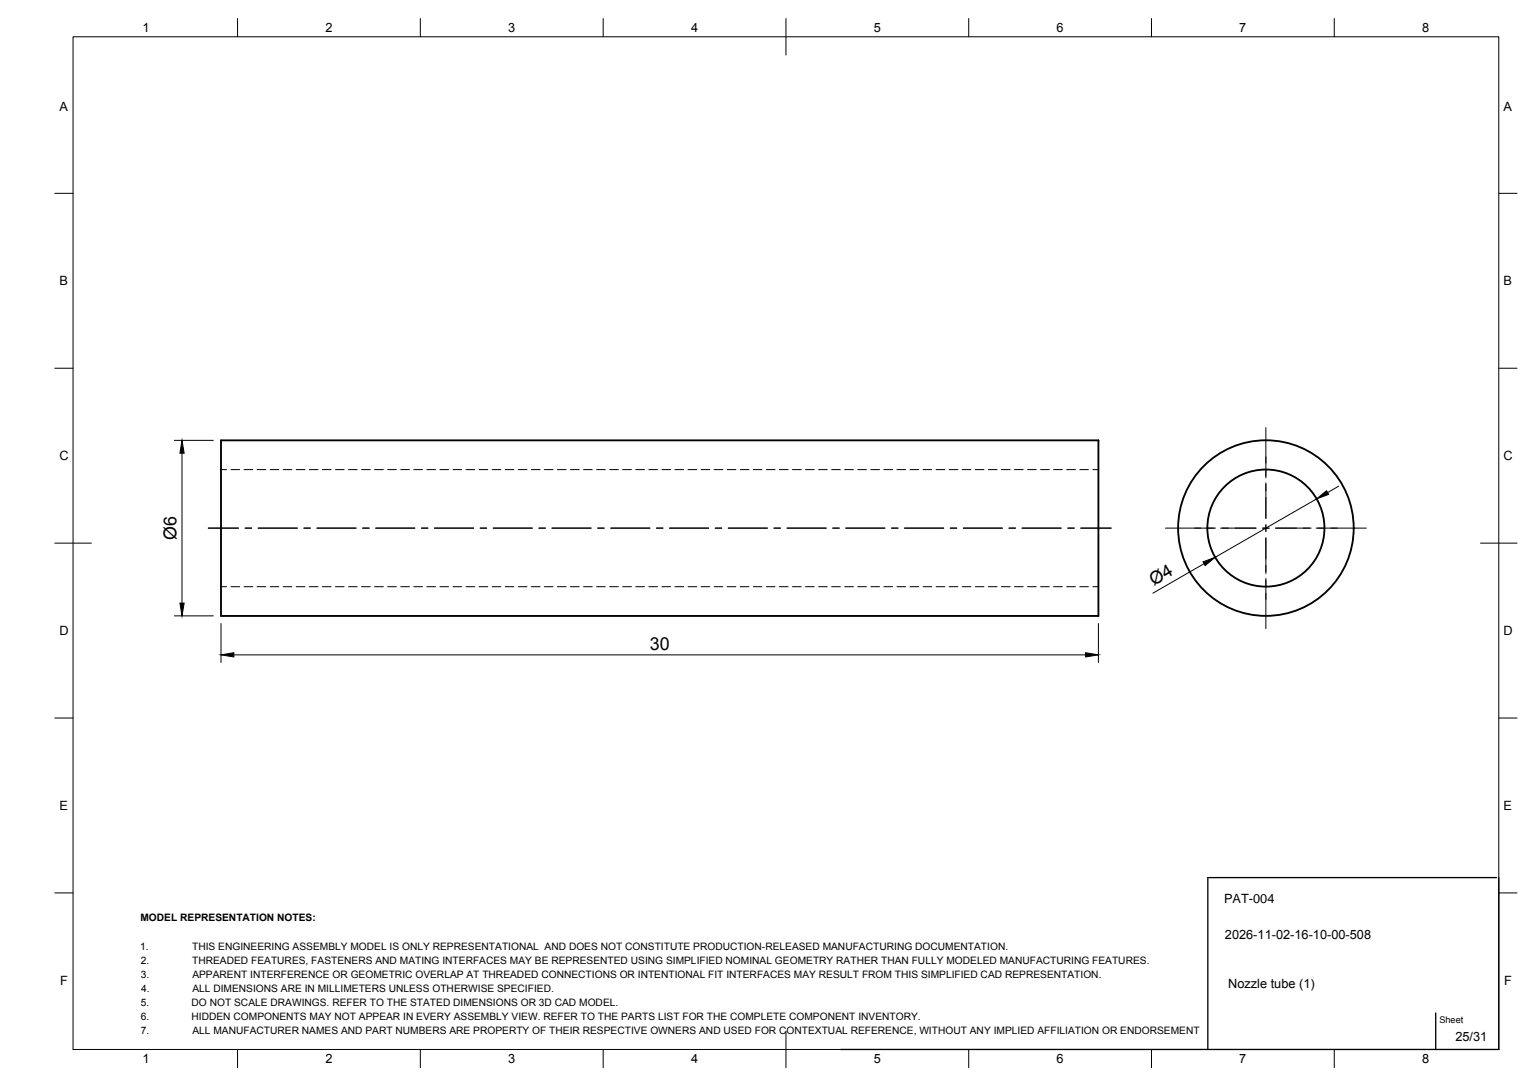
ISO-10303-21;
HEADER;
/* Generated by software containing ST-Developer
 * from STEP Tools, Inc. (www.steptools.com) 
 */

FILE_DESCRIPTION(
/* description */ ('Air blow-off nozzle station'),
/* implementation_level */ '2;1');

FILE_NAME(
/* name */ 'Nozzle tube (1).step',
/* time_stamp */ '2026-10-27T10:53:54-07:00',
/* author */ (''),
/* organization */ (''),
/* preprocessor_version */ 'ST-DEVELOPER v20.2',
/* originating_system */ 'Autodesk Translation Framework v15.17.0.0',
/* authorisation */ '');

FILE_SCHEMA (('AUTOMOTIVE_DESIGN { 1 0 10303 214 3 1 1 }'));
ENDSEC;

DATA;
#10=MECHANICAL_DESIGN_GEOMETRIC_PRESENTATION_REPRESENTATION('',(#255),#7897);
#205=SHAPE_REPRESENTATION_RELATIONSHIP('SRR','None',#8021,#230);
#230=ADVANCED_BREP_SHAPE_REPRESENTATION('',(#278),#7888);
#255=STYLED_ITEM('',(#8206),#278);
#278=MANIFOLD_SOLID_BREP('Body1',#4306);
#348=FACE_BOUND('',#1069,.T.);
#349=FACE_BOUND('',#1071,.T.);
#513=PLANE('',#4960);
#514=PLANE('',#4961);
#747=FACE_OUTER_BOUND('',#1066,.T.);
#748=FACE_OUTER_BOUND('',#1067,.T.);
#749=FACE_OUTER_BOUND('',#1068,.T.);
#750=FACE_OUTER_BOUND('',#1070,.T.);
#1066=EDGE_LOOP('',(#3795,#3796,#3797,#3798));
#1067=EDGE_LOOP('',(#3799,#3800,#3801,#3802));
#1068=EDGE_LOOP('',(#3803));
#1069=EDGE_LOOP('',(#3804));
#1070=EDGE_LOOP('',(#3805));
#1071=EDGE_LOOP('',(#3806));
#1453=LINE('',#7625,#1807);
#1454=LINE('',#7631,#1808);
#1807=VECTOR('',#6121,0.2);
#1808=VECTOR('',#6128,0.3);
#1964=CIRCLE('',#4955,0.2);
#1965=CIRCLE('',#4956,0.2);
#1966=CIRCLE('',#4958,0.3);
#1967=CIRCLE('',#4959,0.3);
#2310=VERTEX_POINT('',#7622);
#2311=VERTEX_POINT('',#7624);
#2312=VERTEX_POINT('',#7628);
#2313=VERTEX_POINT('',#7630);
#2815=EDGE_CURVE('',#2310,#2310,#1964,.T.);
#2816=EDGE_CURVE('',#2310,#2311,#1453,.T.);
#2817=EDGE_CURVE('',#2311,#2311,#1965,.T.);
#2818=EDGE_CURVE('',#2312,#2312,#1966,.T.);
#2819=EDGE_CURVE('',#2312,#2313,#1454,.T.);
#2820=EDGE_CURVE('',#2313,#2313,#1967,.T.);
#3795=ORIENTED_EDGE('',*,*,#2815,.F.);
#3796=ORIENTED_EDGE('',*,*,#2816,.T.);
#3797=ORIENTED_EDGE('',*,*,#2817,.T.);
#3798=ORIENTED_EDGE('',*,*,#2816,.F.);
#3799=ORIENTED_EDGE('',*,*,#2818,.F.);
#3800=ORIENTED_EDGE('',*,*,#2819,.T.);
#3801=ORIENTED_EDGE('',*,*,#2820,.T.);
#3802=ORIENTED_EDGE('',*,*,#2819,.F.);
#3803=ORIENTED_EDGE('',*,*,#2818,.T.);
#3804=ORIENTED_EDGE('',*,*,#2815,.T.);
#3805=ORIENTED_EDGE('',*,*,#2820,.F.);
#3806=ORIENTED_EDGE('',*,*,#2817,.F.);
#4009=CYLINDRICAL_SURFACE('',#4954,0.2);
#4010=CYLINDRICAL_SURFACE('',#4957,0.3);
#4237=ADVANCED_FACE('',(#747),#4009,.F.);
#4238=ADVANCED_FACE('',(#748),#4010,.T.);
#4239=ADVANCED_FACE('',(#749,#348),#513,.T.);
#4240=ADVANCED_FACE('',(#750,#349),#514,.F.);
#4306=CLOSED_SHELL('',(#4237,#4238,#4239,#4240));
#4953=AXIS2_PLACEMENT_3D('',#7620,#6115,#6116);
#4954=AXIS2_PLACEMENT_3D('',#7621,#6117,#6118);
#4955=AXIS2_PLACEMENT_3D('',#7623,#6119,#6120);
#4956=AXIS2_PLACEMENT_3D('',#7626,#6122,#6123);
#4957=AXIS2_PLACEMENT_3D('',#7627,#6124,#6125);
#4958=AXIS2_PLACEMENT_3D('',#7629,#6126,#6127);
#4959=AXIS2_PLACEMENT_3D('',#7632,#6129,#6130);
#4960=AXIS2_PLACEMENT_3D('',#7633,#6131,#6132);
#4961=AXIS2_PLACEMENT_3D('',#7634,#6133,#6134);
#6115=DIRECTION('axis',(0.,0.,1.));
#6116=DIRECTION('refdir',(1.,0.,0.));
#6117=DIRECTION('center_axis',(0.,1.,0.));
#6118=DIRECTION('ref_axis',(1.,0.,0.));
#6119=DIRECTION('center_axis',(0.,-1.,0.));
#6120=DIRECTION('ref_axis',(1.,0.,0.));
#6121=DIRECTION('',(0.,-1.,0.));
#6122=DIRECTION('center_axis',(0.,-1.,0.));
#6123=DIRECTION('ref_axis',(1.,0.,0.));
#6124=DIRECTION('center_axis',(0.,1.,0.));
#6125=DIRECTION('ref_axis',(1.,0.,0.));
#6126=DIRECTION('center_axis',(0.,1.,0.));
#6127=DIRECTION('ref_axis',(1.,0.,0.));
#6128=DIRECTION('',(0.,-1.,0.));
#6129=DIRECTION('center_axis',(0.,1.,0.));
#6130=DIRECTION('ref_axis',(1.,0.,0.));
#6131=DIRECTION('center_axis',(0.,1.,0.));
#6132=DIRECTION('ref_axis',(1.,0.,0.));
#6133=DIRECTION('center_axis',(0.,1.,0.));
#6134=DIRECTION('ref_axis',(1.,0.,0.));
#7620=CARTESIAN_POINT('',(0.,0.,0.));
#7621=CARTESIAN_POINT('Origin',(0.,-7.2,23.));
#7622=CARTESIAN_POINT('',(-0.2,-4.2,23.));
#7623=CARTESIAN_POINT('Origin',(0.,-4.2,23.));
#7624=CARTESIAN_POINT('',(-0.2,-7.2,23.));
#7625=CARTESIAN_POINT('',(-0.2,-7.2,23.));
#7626=CARTESIAN_POINT('Origin',(0.,-7.2,23.));
#7627=CARTESIAN_POINT('Origin',(0.,-7.2,23.));
#7628=CARTESIAN_POINT('',(-0.3,-4.2,23.));
#7629=CARTESIAN_POINT('Origin',(0.,-4.2,23.));
#7630=CARTESIAN_POINT('',(-0.3,-7.2,23.));
#7631=CARTESIAN_POINT('',(-0.3,-7.2,23.));
#7632=CARTESIAN_POINT('Origin',(0.,-7.2,23.));
#7633=CARTESIAN_POINT('Origin',(0.,-4.2,23.));
#7634=CARTESIAN_POINT('Origin',(0.,-7.2,23.));
#7856=UNCERTAINTY_MEASURE_WITH_UNIT(LENGTH_MEASURE(0.001),#7898,
'DISTANCE_ACCURACY_VALUE',
'Maximum model space distance between geometric entities at asserted c
onnectivities');
#7865=UNCERTAINTY_MEASURE_WITH_UNIT(LENGTH_MEASURE(0.001),#7898,
'DISTANCE_ACCURACY_VALUE',
'Maximum model space distance between geometric entities at asserted c
onnectivities');
#7888=(
GEOMETRIC_REPRESENTATION_CONTEXT(3)
GLOBAL_UNCERTAINTY_ASSIGNED_CONTEXT((#7856))
GLOBAL_UNIT_ASSIGNED_CONTEXT((#7898,#7900,#7901))
REPRESENTATION_CONTEXT('','3D')
);
#7897=(
GEOMETRIC_REPRESENTATION_CONTEXT(3)
GLOBAL_UNCERTAINTY_ASSIGNED_CONTEXT((#7865))
GLOBAL_UNIT_ASSIGNED_CONTEXT((#7898,#7900,#7901))
REPRESENTATION_CONTEXT('','3D')
);
#7898=(
LENGTH_UNIT()
NAMED_UNIT(*)
SI_UNIT(.CENTI.,.METRE.)
);
#7900=(
NAMED_UNIT(*)
PLANE_ANGLE_UNIT()
SI_UNIT($,.RADIAN.)
);
#7901=(
NAMED_UNIT(*)
SI_UNIT($,.STERADIAN.)
SOLID_ANGLE_UNIT()
);
#7924=SHAPE_DEFINITION_REPRESENTATION(#7972,#8021);
#7972=PRODUCT_DEFINITION_SHAPE('',$,#8053);
#8021=SHAPE_REPRESENTATION('',(#4953),#7888);
#8030=PRODUCT_DEFINITION_CONTEXT('part definition',#8125,'design');
#8053=PRODUCT_DEFINITION('Nozzle tube (1)','Nozzle tube (1)',#8084,#8030);
#8084=PRODUCT_DEFINITION_FORMATION('',$,#8149);
#8125=APPLICATION_CONTEXT(
'Core Data for Automotive Mechanical Design Process');
#8126=PRODUCT_CONTEXT('part definition',#8125,'mechanical');
#8149=PRODUCT('Nozzle tube (1)','Nozzle tube (1)','Nozzle tube (1)',(#8126));
#8200=COLOUR_RGB('Light Blue',0.38,0.62,0.78);
#8201=FILL_AREA_STYLE_COLOUR('',#8200);
#8202=FILL_AREA_STYLE('',(#8201));
#8203=SURFACE_STYLE_FILL_AREA(#8202);
#8204=SURFACE_SIDE_STYLE('',(#8203));
#8205=SURFACE_STYLE_USAGE(.BOTH.,#8204);
#8206=PRESENTATION_STYLE_ASSIGNMENT((#8205));
ENDSEC;
END-ISO-10303-21;
